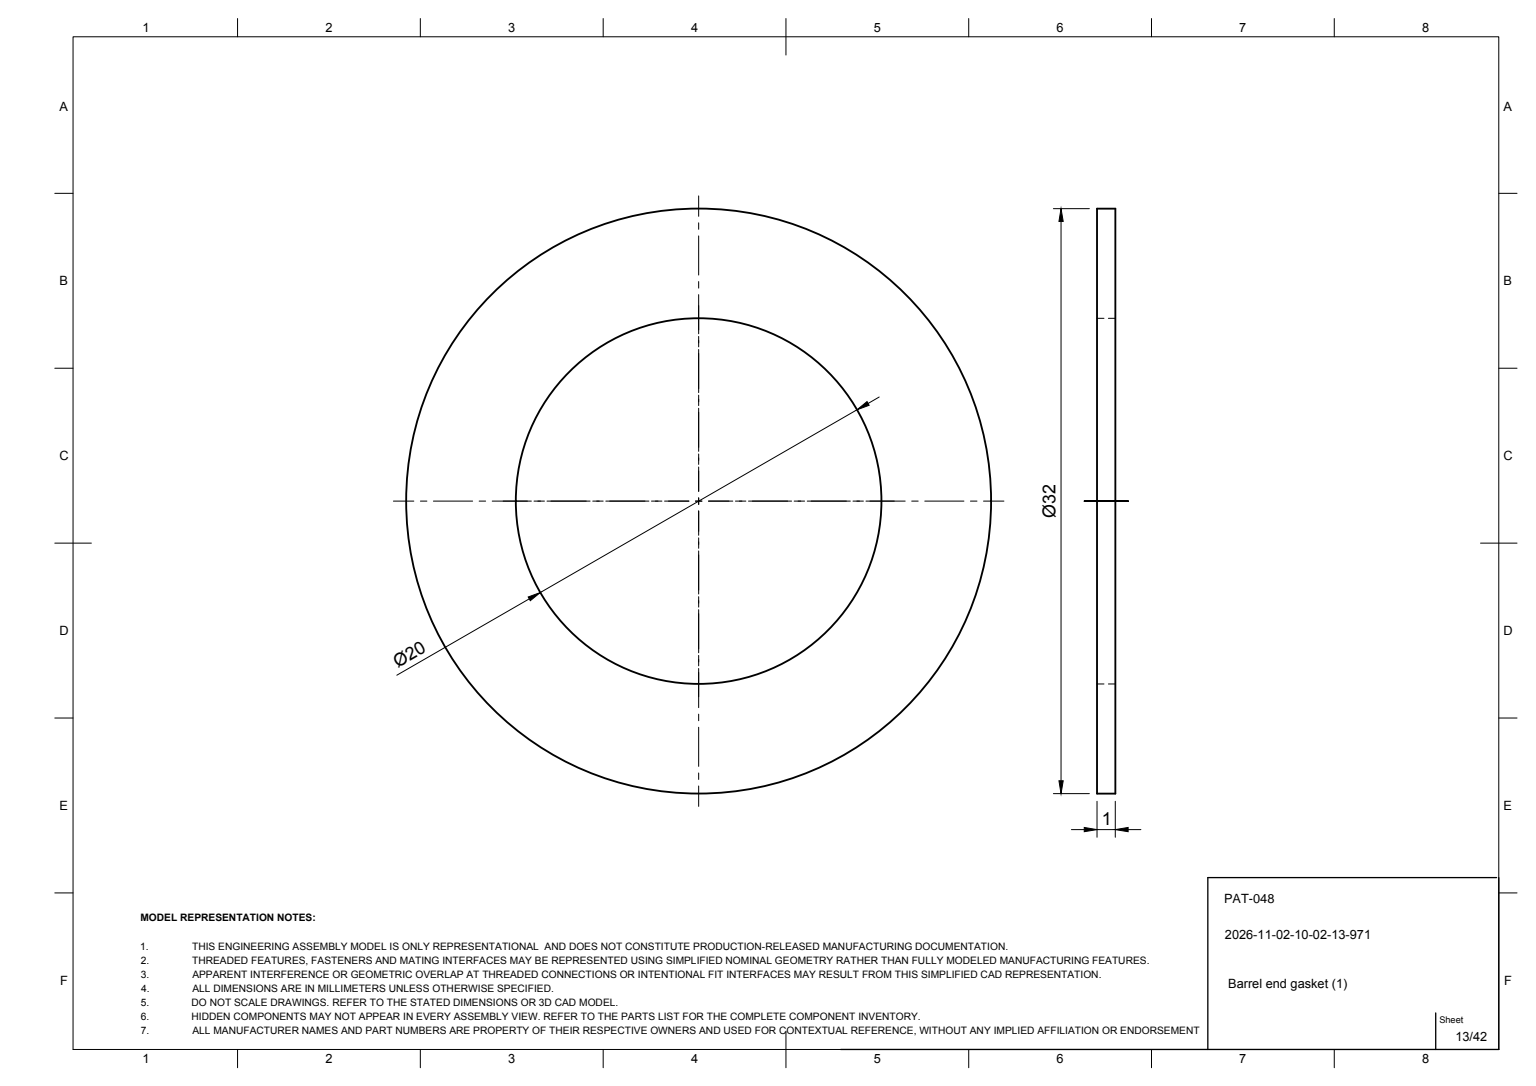
ISO-10303-21;
HEADER;
/* Generated by software containing ST-Developer
 * from STEP Tools, Inc. (www.steptools.com) 
 */

FILE_DESCRIPTION(
/* description */ ('Guided pneumatic stop gate'),
/* implementation_level */ '2;1');

FILE_NAME(
/* name */ 'Barrel end gasket (1).step',
/* time_stamp */ '2026-10-27T21:43:45-07:00',
/* author */ (''),
/* organization */ (''),
/* preprocessor_version */ 'ST-DEVELOPER v20.2',
/* originating_system */ 'Autodesk Translation Framework v15.17.0.0',
/* authorisation */ '');

FILE_SCHEMA (('AUTOMOTIVE_DESIGN { 1 0 10303 214 3 1 1 }'));
ENDSEC;

DATA;
#10=MECHANICAL_DESIGN_GEOMETRIC_PRESENTATION_REPRESENTATION('',(#543),#14392);
#459=SHAPE_REPRESENTATION_RELATIONSHIP('SRR','None',#14593,#501);
#501=ADVANCED_BREP_SHAPE_REPRESENTATION('',(#585),#14355);
#543=STYLED_ITEM('',(#14884),#585);
#585=MANIFOLD_SOLID_BREP('Body1',#7883);
#667=FACE_BOUND('',#1789,.T.);
#668=FACE_BOUND('',#1791,.T.);
#925=PLANE('',#8660);
#926=PLANE('',#8661);
#1259=FACE_OUTER_BOUND('',#1786,.T.);
#1260=FACE_OUTER_BOUND('',#1787,.T.);
#1261=FACE_OUTER_BOUND('',#1788,.T.);
#1262=FACE_OUTER_BOUND('',#1790,.T.);
#1786=EDGE_LOOP('',(#5886,#5887,#5888,#5889));
#1787=EDGE_LOOP('',(#5890,#5891,#5892,#5893));
#1788=EDGE_LOOP('',(#5894));
#1789=EDGE_LOOP('',(#5895));
#1790=EDGE_LOOP('',(#5896));
#1791=EDGE_LOOP('',(#5897));
#2445=LINE('',#12539,#2990);
#2446=LINE('',#12545,#2991);
#2990=VECTOR('',#10092,1.);
#2991=VECTOR('',#10099,1.6);
#3472=CIRCLE('',#8655,1.);
#3473=CIRCLE('',#8656,1.);
#3474=CIRCLE('',#8658,1.6);
#3475=CIRCLE('',#8659,1.6);
#3915=VERTEX_POINT('',#12536);
#3916=VERTEX_POINT('',#12538);
#3917=VERTEX_POINT('',#12542);
#3918=VERTEX_POINT('',#12544);
#4641=EDGE_CURVE('',#3915,#3915,#3472,.T.);
#4642=EDGE_CURVE('',#3915,#3916,#2445,.T.);
#4643=EDGE_CURVE('',#3916,#3916,#3473,.T.);
#4644=EDGE_CURVE('',#3917,#3917,#3474,.T.);
#4645=EDGE_CURVE('',#3917,#3918,#2446,.T.);
#4646=EDGE_CURVE('',#3918,#3918,#3475,.T.);
#5886=ORIENTED_EDGE('',*,*,#4641,.F.);
#5887=ORIENTED_EDGE('',*,*,#4642,.T.);
#5888=ORIENTED_EDGE('',*,*,#4643,.T.);
#5889=ORIENTED_EDGE('',*,*,#4642,.F.);
#5890=ORIENTED_EDGE('',*,*,#4644,.F.);
#5891=ORIENTED_EDGE('',*,*,#4645,.T.);
#5892=ORIENTED_EDGE('',*,*,#4646,.T.);
#5893=ORIENTED_EDGE('',*,*,#4645,.F.);
#5894=ORIENTED_EDGE('',*,*,#4644,.T.);
#5895=ORIENTED_EDGE('',*,*,#4641,.T.);
#5896=ORIENTED_EDGE('',*,*,#4646,.F.);
#5897=ORIENTED_EDGE('',*,*,#4643,.F.);
#7287=CYLINDRICAL_SURFACE('',#8654,1.);
#7288=CYLINDRICAL_SURFACE('',#8657,1.6);
#7541=ADVANCED_FACE('',(#1259),#7287,.F.);
#7542=ADVANCED_FACE('',(#1260),#7288,.T.);
#7543=ADVANCED_FACE('',(#1261,#667),#925,.T.);
#7544=ADVANCED_FACE('',(#1262,#668),#926,.F.);
#7883=CLOSED_SHELL('',(#7541,#7542,#7543,#7544));
#8653=AXIS2_PLACEMENT_3D('',#12534,#10086,#10087);
#8654=AXIS2_PLACEMENT_3D('',#12535,#10088,#10089);
#8655=AXIS2_PLACEMENT_3D('',#12537,#10090,#10091);
#8656=AXIS2_PLACEMENT_3D('',#12540,#10093,#10094);
#8657=AXIS2_PLACEMENT_3D('',#12541,#10095,#10096);
#8658=AXIS2_PLACEMENT_3D('',#12543,#10097,#10098);
#8659=AXIS2_PLACEMENT_3D('',#12546,#10100,#10101);
#8660=AXIS2_PLACEMENT_3D('',#12547,#10102,#10103);
#8661=AXIS2_PLACEMENT_3D('',#12548,#10104,#10105);
#10086=DIRECTION('axis',(0.,0.,1.));
#10087=DIRECTION('refdir',(1.,0.,0.));
#10088=DIRECTION('center_axis',(0.,1.,0.));
#10089=DIRECTION('ref_axis',(1.,0.,0.));
#10090=DIRECTION('center_axis',(0.,-1.,0.));
#10091=DIRECTION('ref_axis',(1.,0.,0.));
#10092=DIRECTION('',(0.,-1.,0.));
#10093=DIRECTION('center_axis',(0.,-1.,0.));
#10094=DIRECTION('ref_axis',(1.,0.,0.));
#10095=DIRECTION('center_axis',(0.,1.,0.));
#10096=DIRECTION('ref_axis',(1.,0.,0.));
#10097=DIRECTION('center_axis',(0.,1.,0.));
#10098=DIRECTION('ref_axis',(1.,0.,0.));
#10099=DIRECTION('',(0.,-1.,0.));
#10100=DIRECTION('center_axis',(0.,1.,0.));
#10101=DIRECTION('ref_axis',(1.,0.,0.));
#10102=DIRECTION('center_axis',(0.,1.,0.));
#10103=DIRECTION('ref_axis',(1.,0.,0.));
#10104=DIRECTION('center_axis',(0.,1.,0.));
#10105=DIRECTION('ref_axis',(1.,0.,0.));
#12534=CARTESIAN_POINT('',(0.,0.,0.));
#12535=CARTESIAN_POINT('Origin',(0.,10.8,4.5));
#12536=CARTESIAN_POINT('',(-1.,10.9,4.5));
#12537=CARTESIAN_POINT('Origin',(0.,10.9,4.5));
#12538=CARTESIAN_POINT('',(-1.,10.8,4.5));
#12539=CARTESIAN_POINT('',(-1.,10.8,4.5));
#12540=CARTESIAN_POINT('Origin',(0.,10.8,4.5));
#12541=CARTESIAN_POINT('Origin',(0.,10.8,4.5));
#12542=CARTESIAN_POINT('',(-1.6,10.9,4.5));
#12543=CARTESIAN_POINT('Origin',(0.,10.9,4.5));
#12544=CARTESIAN_POINT('',(-1.6,10.8,4.5));
#12545=CARTESIAN_POINT('',(-1.6,10.8,4.5));
#12546=CARTESIAN_POINT('Origin',(0.,10.8,4.5));
#12547=CARTESIAN_POINT('Origin',(0.,10.9,4.5));
#12548=CARTESIAN_POINT('Origin',(0.,10.8,4.5));
#14307=UNCERTAINTY_MEASURE_WITH_UNIT(LENGTH_MEASURE(0.001),#14393,
'DISTANCE_ACCURACY_VALUE',
'Maximum model space distance between geometric entities at asserted c
onnectivities');
#14344=UNCERTAINTY_MEASURE_WITH_UNIT(LENGTH_MEASURE(0.001),#14393,
'DISTANCE_ACCURACY_VALUE',
'Maximum model space distance between geometric entities at asserted c
onnectivities');
#14355=(
GEOMETRIC_REPRESENTATION_CONTEXT(3)
GLOBAL_UNCERTAINTY_ASSIGNED_CONTEXT((#14307))
GLOBAL_UNIT_ASSIGNED_CONTEXT((#14393,#14395,#14396))
REPRESENTATION_CONTEXT('','3D')
);
#14392=(
GEOMETRIC_REPRESENTATION_CONTEXT(3)
GLOBAL_UNCERTAINTY_ASSIGNED_CONTEXT((#14344))
GLOBAL_UNIT_ASSIGNED_CONTEXT((#14393,#14395,#14396))
REPRESENTATION_CONTEXT('','3D')
);
#14393=(
LENGTH_UNIT()
NAMED_UNIT(*)
SI_UNIT(.CENTI.,.METRE.)
);
#14395=(
NAMED_UNIT(*)
PLANE_ANGLE_UNIT()
SI_UNIT($,.RADIAN.)
);
#14396=(
NAMED_UNIT(*)
SI_UNIT($,.STERADIAN.)
SOLID_ANGLE_UNIT()
);
#14407=SHAPE_DEFINITION_REPRESENTATION(#14454,#14593);
#14454=PRODUCT_DEFINITION_SHAPE('',$,#14641);
#14593=SHAPE_REPRESENTATION('',(#8653),#14355);
#14630=PRODUCT_DEFINITION_CONTEXT('part definition',#14773,'design');
#14641=PRODUCT_DEFINITION('Barrel end gasket (1)','Barrel end gasket (1)',
#14688,#14630);
#14688=PRODUCT_DEFINITION_FORMATION('',$,#14785);
#14773=APPLICATION_CONTEXT(
'Core Data for Automotive Mechanical Design Process');
#14774=PRODUCT_CONTEXT('part definition',#14773,'mechanical');
#14785=PRODUCT('Barrel end gasket (1)','Barrel end gasket (1)',
'Barrel end gasket (1)',(#14774));
#14878=COLOUR_RGB('Sky Blue',0.24,0.69,0.87);
#14879=FILL_AREA_STYLE_COLOUR('',#14878);
#14880=FILL_AREA_STYLE('',(#14879));
#14881=SURFACE_STYLE_FILL_AREA(#14880);
#14882=SURFACE_SIDE_STYLE('',(#14881));
#14883=SURFACE_STYLE_USAGE(.BOTH.,#14882);
#14884=PRESENTATION_STYLE_ASSIGNMENT((#14883));
ENDSEC;
END-ISO-10303-21;
